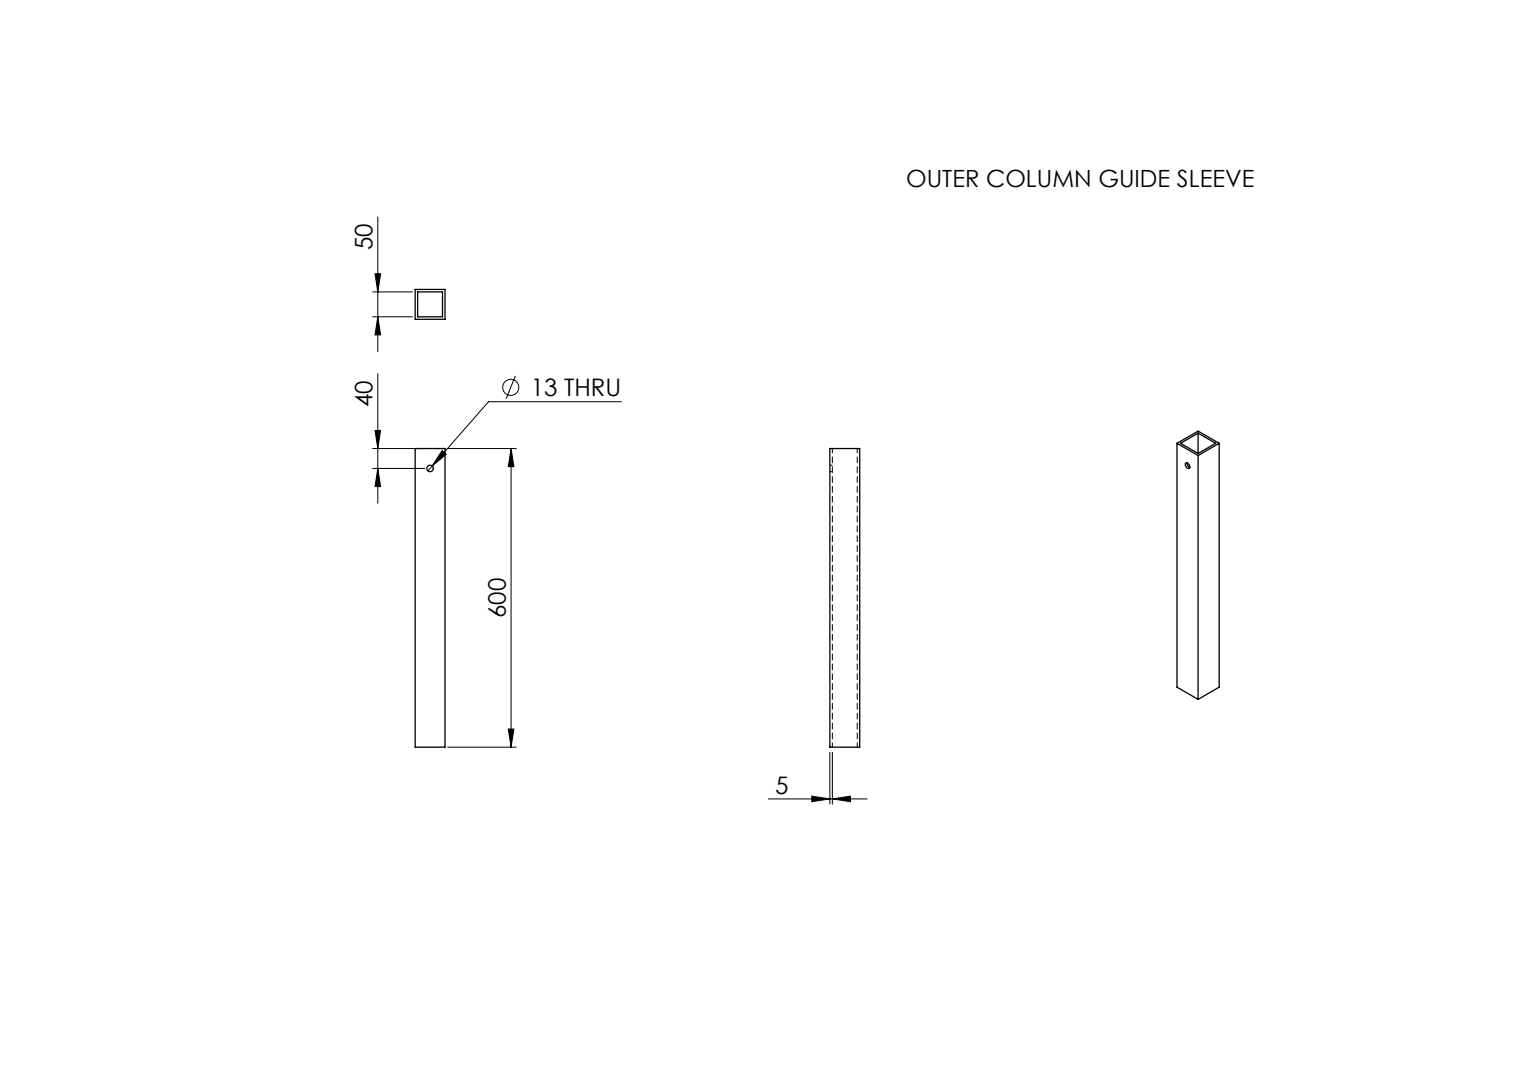
ISO-10303-21;
HEADER;
FILE_DESCRIPTION (('STEP AP214'),
    '1' );
FILE_NAME ('Outer Column Guide Sleeve.step',
    '2026-10-22T16:49:52',
    ( '' ),
    ( '' ),
    'SwSTEP 2.0',
    'SolidWorks 2026',
    '' );
FILE_SCHEMA (( 'AUTOMOTIVE_DESIGN' ));
ENDSEC;

DATA;
#4=( LENGTH_UNIT ( ) NAMED_UNIT ( * ) SI_UNIT ( .MILLI., .METRE. ) );
#55=DIRECTION ( 'NONE',  ( 0.000000000000000000, -0.000000000000000000, 1.000000000000000000 ) ) ;
#57=LINE ( 'NONE', #1683, #3118 ) ;
#59=CIRCLE ( 'NONE', #3730, 6.499999999999983125 ) ;
#64=DIRECTION ( 'NONE',  ( -0.000000000000000000, -0.000000000000000000, 1.000000000000000000 ) ) ;
#65=LINE ( 'NONE', #137, #1780 ) ;
#71=EDGE_LOOP ( 'NONE', ( #1973, #4142, #2111, #5305 ) ) ;
#74=DIRECTION ( 'NONE',  ( 1.000000000000000000, 0.000000000000000000, 0.000000000000000000 ) ) ;
#78=DIRECTION ( 'NONE',  ( -6.938893903907228378E-17, 0.000000000000000000, 1.000000000000000000 ) ) ;
#82=ORIENTED_EDGE ( 'NONE', *, *, #2566, .T. ) ;
#104=MANIFOLD_SOLID_BREP ( 'M12 Clearance Hole1', #2049 ) ;
#118=CIRCLE ( 'NONE', #3006, 6.499999999999988454 ) ;
#134=CARTESIAN_POINT ( 'NONE',  ( 30.00000000000000355, 610.0000000000000000, 30.00000000000001066 ) ) ;
#137=CARTESIAN_POINT ( 'NONE',  ( -24.99999999999999645, 610.0000000000000000, -25.00000000000000000 ) ) ;
#144=CARTESIAN_POINT ( 'NONE',  ( 0.000000000000000000, 570.0000000000000000, 25.00000000000000000 ) ) ;
#145=VECTOR ( 'NONE', #5158, 1000.000000000000000 ) ;
#150=VECTOR ( 'NONE', #4769, 1000.000000000000000 ) ;
#169=ORIENTED_EDGE ( 'NONE', *, *, #1169, .T. ) ;
#177=ORIENTED_EDGE ( 'NONE', *, *, #2712, .T. ) ;
#203=DIRECTION ( 'NONE',  ( 0.000000000000000000, 0.000000000000000000, -1.000000000000000000 ) ) ;
#213=DIRECTION ( 'NONE',  ( -1.000000000000000000, 0.000000000000000000, -2.081668171172168513E-16 ) ) ;
#220=ORIENTED_EDGE ( 'NONE', *, *, #4751, .F. ) ;
#236=CYLINDRICAL_SURFACE ( 'NONE', #2573, 6.499999999999983125 ) ;
#257=CARTESIAN_POINT ( 'NONE',  ( 30.00000000000000355, 610.0000000000000000, 30.00000000000001066 ) ) ;
#293=FACE_OUTER_BOUND ( 'NONE', #4919, .T. ) ;
#296=ORIENTED_EDGE ( 'NONE', *, *, #4163, .F. ) ;
#299=DIRECTION ( 'NONE',  ( -0.000000000000000000, -0.000000000000000000, 1.000000000000000000 ) ) ;
#306=DIRECTION ( 'NONE',  ( 1.000000000000000000, 0.000000000000000000, -0.000000000000000000 ) ) ;
#311=DIRECTION ( 'NONE',  ( -0.000000000000000000, -0.000000000000000000, 1.000000000000000000 ) ) ;
#324=EDGE_LOOP ( 'NONE', ( #2487, #2510, #2629, #3709 ) ) ;
#333=DIRECTION ( 'NONE',  ( -0.000000000000000000, -0.000000000000000000, 1.000000000000000000 ) ) ;
#337=FACE_OUTER_BOUND ( 'NONE', #718, .T. ) ;
#345=CARTESIAN_POINT ( 'NONE',  ( 30.00000000000000355, 610.0000000000000000, 0.000000000000000000 ) ) ;
#347=ORIENTED_EDGE ( 'NONE', *, *, #1984, .F. ) ;
#348=EDGE_LOOP ( 'NONE', ( #4253, #4137 ) ) ;
#363=FACE_BOUND ( 'NONE', #348, .T. ) ;
#384=ORIENTED_EDGE ( 'NONE', *, *, #564, .F. ) ;
#386=CARTESIAN_POINT ( 'NONE',  ( -30.00000000000000355, 610.0000000000000000, -2.081668171172168908E-15 ) ) ;
#401=( GEOMETRIC_REPRESENTATION_CONTEXT ( 3 ) GLOBAL_UNCERTAINTY_ASSIGNED_CONTEXT ( ( #3253 ) ) GLOBAL_UNIT_ASSIGNED_CONTEXT ( ( #4, #2110, #4596 ) ) REPRESENTATION_CONTEXT ( 'NONE', 'WORKASPACE' ) );
#441=CARTESIAN_POINT ( 'NONE',  ( -1.676835913137321903E-15, 35.00000000000000000, -25.00000000000000000 ) ) ;
#445=ORIENTED_EDGE ( 'NONE', *, *, #3007, .T. ) ;
#474=ORIENTED_EDGE ( 'NONE', *, *, #2211, .F. ) ;
#494=VECTOR ( 'NONE', #4759, 1000.000000000000000 ) ;
#502=AXIS2_PLACEMENT_3D ( 'NONE', #1265, #2612, #74 ) ;
#505=DIRECTION ( 'NONE',  ( -0.000000000000000000, -0.000000000000000000, 1.000000000000000000 ) ) ;
#516=DIRECTION ( 'NONE',  ( -0.000000000000000000, -1.000000000000000000, -0.000000000000000000 ) ) ;
#522=LINE ( 'NONE', #1310, #5104 ) ;
#525=ORIENTED_EDGE ( 'NONE', *, *, #1984, .T. ) ;
#528=CARTESIAN_POINT ( 'NONE',  ( -24.99999999999999645, 610.0000000000000000, -25.00000000000000000 ) ) ;
#536=DIRECTION ( 'NONE',  ( -0.000000000000000000, -0.000000000000000000, 1.000000000000000000 ) ) ;
#554=CARTESIAN_POINT ( 'NONE',  ( -1.676835913137321903E-15, 35.00000000000000000, 30.00000000000000711 ) ) ;
#555=CIRCLE ( 'NONE', #1685, 6.499999999999983125 ) ;
#564=EDGE_CURVE ( 'NONE', #1204, #676, #3614, .T. ) ;
#568=ORIENTED_EDGE ( 'NONE', *, *, #2743, .T. ) ;
#591=CARTESIAN_POINT ( 'NONE',  ( 0.000000000000000000, 570.0000000000000000, 25.00000000000000000 ) ) ;
#615=EDGE_LOOP ( 'NONE', ( #2413, #3333, #5322, #568 ) ) ;
#635=ORIENTED_EDGE ( 'NONE', *, *, #2387, .T. ) ;
#639=ORIENTED_EDGE ( 'NONE', *, *, #709, .F. ) ;
#652=VECTOR ( 'NONE', #4092, 1000.000000000000000 ) ;
#659=CARTESIAN_POINT ( 'NONE',  ( -24.99999999999999645, 610.0000000000000000, -25.00000000000000000 ) ) ;
#674=EDGE_LOOP ( 'NONE', ( #474, #4449, #1677, #4999 ) ) ;
#676=VERTEX_POINT ( 'NONE', #2760 ) ;
#680=VECTOR ( 'NONE', #5152, 1000.000000000000000 ) ;
#681=ORIENTED_EDGE ( 'NONE', *, *, #2414, .T. ) ;
#684=CARTESIAN_POINT ( 'NONE',  ( -30.00000000000000000, 610.0000000000000000, -30.00000000000000355 ) ) ;
#706=DIRECTION ( 'NONE',  ( 0.000000000000000000, -0.000000000000000000, 1.000000000000000000 ) ) ;
#709=EDGE_CURVE ( 'NONE', #819, #4789, #1060, .T. ) ;
#714=DIRECTION ( 'NONE',  ( -1.000000000000000000, 0.000000000000000000, -0.000000000000000000 ) ) ;
#718=EDGE_LOOP ( 'NONE', ( #2881, #2906, #4894, #4616 ) ) ;
#722=LINE ( 'NONE', #5277, #1209 ) ;
#734=AXIS2_PLACEMENT_3D ( 'NONE', #3221, #1943, #706 ) ;
#735=ORIENTED_EDGE ( 'NONE', *, *, #1905, .T. ) ;
#751=COLOUR_RGB ( '',0.8941176470588234615, 0.8941176470588234615, 0.8941176470588234615 ) ;
#761=VECTOR ( 'NONE', #2328, 1000.000000000000000 ) ;
#767=ORIENTED_EDGE ( 'NONE', *, *, #3722, .F. ) ;
#769=DIRECTION ( 'NONE',  ( 1.000000000000000000, 0.000000000000000000, 0.000000000000000000 ) ) ;
#776=DIRECTION ( 'NONE',  ( 1.000000000000000000, 0.000000000000000000, 0.000000000000000000 ) ) ;
#797=CARTESIAN_POINT ( 'NONE',  ( 25.00000000000000000, 610.0000000000000000, 25.00000000000000711 ) ) ;
#819=VERTEX_POINT ( 'NONE', #797 ) ;
#823=DIRECTION ( 'NONE',  ( -1.000000000000000000, 0.000000000000000000, 0.000000000000000000 ) ) ;
#834=LINE ( 'NONE', #4115, #1093 ) ;
#840=PRODUCT_DEFINITION_FORMATION_WITH_SPECIFIED_SOURCE ( 'ANY', '', #918, .NOT_KNOWN. ) ;
#845=FILL_AREA_STYLE ('',( #3720 ) ) ;
#851=EDGE_LOOP ( 'NONE', ( #978, #1701, #2976, #2915 ) ) ;
#858=CARTESIAN_POINT ( 'NONE',  ( 0.000000000000000000, 570.0000000000000000, 30.00000000000000711 ) ) ;
#868=FACE_OUTER_BOUND ( 'NONE', #5245, .T. ) ;
#890=CARTESIAN_POINT ( 'NONE',  ( -1.676835913137321903E-15, 35.00000000000000000, -30.00000000000000711 ) ) ;
#911=ADVANCED_FACE ( 'NONE', ( #2175 ), #2619, .T. ) ;
#918=PRODUCT ( 'Outer Column Guide Sleeve', 'Outer Column Guide Sleeve', '', ( #3228 ) ) ;
#927=ORIENTED_EDGE ( 'NONE', *, *, #4973, .F. ) ;
#933=( NAMED_UNIT ( * ) SI_UNIT ( $, .STERADIAN. ) SOLID_ANGLE_UNIT ( ) );
#939=DIRECTION ( 'NONE',  ( -0.000000000000000000, -0.000000000000000000, 1.000000000000000000 ) ) ;
#966=VERTEX_POINT ( 'NONE', #3415 ) ;
#969=CARTESIAN_POINT ( 'NONE',  ( 25.00000000000000000, 610.0000000000000000, 25.00000000000000711 ) ) ;
#978=ORIENTED_EDGE ( 'NONE', *, *, #1193, .T. ) ;
#984=LINE ( 'NONE', #1407, #145 ) ;
#995=DIRECTION ( 'NONE',  ( -0.000000000000000000, -1.000000000000000000, -0.000000000000000000 ) ) ;
#1021=EDGE_CURVE ( 'NONE', #1591, #4832, #555, .T. ) ;
#1038=DIRECTION ( 'NONE',  ( 0.000000000000000000, 0.000000000000000000, -1.000000000000000000 ) ) ;
#1040=PLANE ( 'NONE',  #3295 ) ;
#1049=CARTESIAN_POINT ( 'NONE',  ( -30.00000000000000355, 610.0000000000000000, 30.00000000000000000 ) ) ;
#1054=ORIENTED_EDGE ( 'NONE', *, *, #4694, .T. ) ;
#1060=LINE ( 'NONE', #4411, #5259 ) ;
#1061=LINE ( 'NONE', #2731, #2423 ) ;
#1062=FACE_BOUND ( 'NONE', #2196, .T. ) ;
#1065=SHAPE_REPRESENTATION ( 'Outer Column Guide Sleeve', ( #4154 ), #3189 ) ;
#1066=EDGE_CURVE ( 'NONE', #2454, #4719, #118, .T. ) ;
#1069=CARTESIAN_POINT ( 'NONE',  ( 30.00000000000000355, 610.0000000000000000, 0.000000000000000000 ) ) ;
#1074=CARTESIAN_POINT ( 'NONE',  ( -25.00000000000000000, 610.0000000000000000, 24.99999999999999645 ) ) ;
#1075=VERTEX_POINT ( 'NONE', #5044 ) ;
#1093=VECTOR ( 'NONE', #4947, 1000.000000000000000 ) ;
#1101=AXIS2_PLACEMENT_3D ( 'NONE', #1578, #5333, #3322 ) ;
#1105=FACE_OUTER_BOUND ( 'NONE', #71, .T. ) ;
#1109=EDGE_CURVE ( 'NONE', #3821, #4454, #1453, .T. ) ;
#1122=UNCERTAINTY_MEASURE_WITH_UNIT (LENGTH_MEASURE( 1.000000000000000082E-05 ), #3066, 'distance_accuracy_value', 'NONE');
#1124=EDGE_LOOP ( 'NONE', ( #2187, #2700, #3235, #525 ) ) ;
#1125=PLANE ( 'NONE',  #3717 ) ;
#1138=PLANE ( 'NONE',  #734 ) ;
#1169=EDGE_CURVE ( 'NONE', #4363, #3498, #2834, .T. ) ;
#1193=EDGE_CURVE ( 'NONE', #1510, #1969, #3155, .T. ) ;
#1199=CARTESIAN_POINT ( 'NONE',  ( 30.00000000000000355, 10.00000000000000000, -30.00000000000000355 ) ) ;
#1203=( NAMED_UNIT ( * ) PLANE_ANGLE_UNIT ( ) SI_UNIT ( $, .RADIAN. ) );
#1204=VERTEX_POINT ( 'NONE', #1393 ) ;
#1209=VECTOR ( 'NONE', #311, 1000.000000000000000 ) ;
#1228=SHAPE_REPRESENTATION_RELATIONSHIP ( 'NONE' , 'NONE' ,  #1065, #4286 ) ;
#1241=EDGE_CURVE ( 'NONE', #4454, #966, #3104, .T. ) ;
#1249=EDGE_LOOP ( 'NONE', ( #767, #2867, #5272, #681 ) ) ;
#1265=CARTESIAN_POINT ( 'NONE',  ( -1.676835913137321903E-15, 35.00000000000000000, -25.00000000000000000 ) ) ;
#1275=ADVANCED_FACE ( 'NONE', ( #5288, #4865 ), #1138, .T. ) ;
#1283=AXIS2_PLACEMENT_3D ( 'NONE', #3128, #4799, #3416 ) ;
#1285=ORIENTED_EDGE ( 'NONE', *, *, #3872, .F. ) ;
#1294=ORIENTED_EDGE ( 'NONE', *, *, #4878, .T. ) ;
#1310=CARTESIAN_POINT ( 'NONE',  ( -6.245004513516506329E-15, 610.0000000000000000, 30.00000000000000711 ) ) ;
#1317=DIRECTION ( 'NONE',  ( 1.000000000000000000, 0.000000000000000000, 0.000000000000000000 ) ) ;
#1348=DIRECTION ( 'NONE',  ( -0.000000000000000000, -1.000000000000000000, -0.000000000000000000 ) ) ;
#1358=DIRECTION ( 'NONE',  ( -1.000000000000000000, 0.000000000000000000, 0.000000000000000000 ) ) ;
#1366=DIRECTION ( 'NONE',  ( -1.000000000000000000, 0.000000000000000000, 0.000000000000000000 ) ) ;
#1374=DIRECTION ( 'NONE',  ( 6.938893903907228378E-17, 0.000000000000000000, -1.000000000000000000 ) ) ;
#1384=DIRECTION ( 'NONE',  ( 2.081668171172168513E-16, 0.000000000000000000, -1.000000000000000000 ) ) ;
#1393=CARTESIAN_POINT ( 'NONE',  ( -6.499999999999984901, 35.00000000000000000, 25.00000000000000000 ) ) ;
#1397=VERTEX_POINT ( 'NONE', #2602 ) ;
#1407=CARTESIAN_POINT ( 'NONE',  ( 30.00000000000000355, 610.0000000000000000, -30.00000000000000355 ) ) ;
#1410=FACE_OUTER_BOUND ( 'NONE', #1249, .T. ) ;
#1414=VECTOR ( 'NONE', #1348, 1000.000000000000000 ) ;
#1453=LINE ( 'NONE', #2226, #3873 ) ;
#1457=VERTEX_POINT ( 'NONE', #4315 ) ;
#1468=CARTESIAN_POINT ( 'NONE',  ( 25.00000000000000000, 10.00000000000000000, -25.00000000000000000 ) ) ;
#1478=EDGE_LOOP ( 'NONE', ( #4056, #1960 ) ) ;
#1483=ORIENTED_EDGE ( 'NONE', *, *, #3142, .T. ) ;
#1503=AXIS2_PLACEMENT_3D ( 'NONE', #591, #3185, #4780 ) ;
#1509=ADVANCED_FACE ( 'NONE', ( #5106, #2689 ), #4345, .F. ) ;
#1510=VERTEX_POINT ( 'NONE', #5156 ) ;
#1511=VECTOR ( 'NONE', #78, 1000.000000000000000 ) ;
#1532=ORIENTED_EDGE ( 'NONE', *, *, #5162, .T. ) ;
#1534=VECTOR ( 'NONE', #4371, 1000.000000000000000 ) ;
#1578=CARTESIAN_POINT ( 'NONE',  ( -6.245004513516506329E-15, 610.0000000000000000, 30.00000000000000711 ) ) ;
#1591=VERTEX_POINT ( 'NONE', #3674 ) ;
#1601=AXIS2_PLACEMENT_3D ( 'NONE', #3718, #3746, #5371 ) ;
#1619=AXIS2_PLACEMENT_3D ( 'NONE', #386, #2917, #2497 ) ;
#1626=( LENGTH_UNIT ( ) NAMED_UNIT ( * ) SI_UNIT ( .MILLI., .METRE. ) );
#1653=ADVANCED_FACE ( 'NONE', ( #4851, #337 ), #1125, .F. ) ;
#1657=ORIENTED_EDGE ( 'NONE', *, *, #5072, .T. ) ;
#1665=( GEOMETRIC_REPRESENTATION_CONTEXT ( 3 ) GLOBAL_UNCERTAINTY_ASSIGNED_CONTEXT ( ( #1122 ) ) GLOBAL_UNIT_ASSIGNED_CONTEXT ( ( #3066, #4242, #933 ) ) REPRESENTATION_CONTEXT ( 'NONE', 'WORKASPACE' ) );
#1677=ORIENTED_EDGE ( 'NONE', *, *, #4751, .T. ) ;
#1678=ORIENTED_EDGE ( 'NONE', *, *, #3048, .T. ) ;
#1683=CARTESIAN_POINT ( 'NONE',  ( 6.499999999999981348, 35.00000000000000000, 30.00000000000000711 ) ) ;
#1685=AXIS2_PLACEMENT_3D ( 'NONE', #890, #55, #4643 ) ;
#1688=AXIS2_PLACEMENT_3D ( 'NONE', #4682, #1828, #4287 ) ;
#1690=FACE_OUTER_BOUND ( 'NONE', #2461, .T. ) ;
#1697=PLANE ( 'NONE',  #2774 ) ;
#1701=ORIENTED_EDGE ( 'NONE', *, *, #3430, .F. ) ;
#1713=DIRECTION ( 'NONE',  ( 1.000000000000000000, 0.000000000000000000, 0.000000000000000000 ) ) ;
#1718=EDGE_CURVE ( 'NONE', #4147, #4026, #4642, .T. ) ;
#1727=AXIS2_PLACEMENT_3D ( 'NONE', #2764, #333, #4108 ) ;
#1750=STYLED_ITEM('',(#5440),#104);
#1758=CARTESIAN_POINT ( 'NONE',  ( -25.00000000000000000, 610.0000000000000000, 24.99999999999999645 ) ) ;
#1765=CARTESIAN_POINT ( 'NONE',  ( -1.676835913137321903E-15, 35.00000000000000000, 25.00000000000000000 ) ) ;
#1770=ORIENTED_EDGE ( 'NONE', *, *, #1109, .T. ) ;
#1780=VECTOR ( 'NONE', #1825, 1000.000000000000000 ) ;
#1801=ORIENTED_EDGE ( 'NONE', *, *, #4432, .T. ) ;
#1815=ADVANCED_FACE ( 'NONE', ( #4330 ), #236, .F. ) ;
#1823=DIRECTION ( 'NONE',  ( -1.000000000000000000, 0.000000000000000000, 0.000000000000000000 ) ) ;
#1825=DIRECTION ( 'NONE',  ( -1.000000000000000000, 0.000000000000000000, -0.000000000000000000 ) ) ;
#1828=DIRECTION ( 'NONE',  ( 0.000000000000000000, 1.000000000000000000, 0.000000000000000000 ) ) ;
#1872=CARTESIAN_POINT ( 'NONE',  ( 6.499999999999981348, 35.00000000000000000, -30.00000000000000711 ) ) ;
#1883=CARTESIAN_POINT ( 'NONE',  ( -6.499999999999984901, 35.00000000000000000, -25.00000000000000000 ) ) ;
#1890=VECTOR ( 'NONE', #516, 1000.000000000000000 ) ;
#1895=CARTESIAN_POINT ( 'NONE',  ( 0.000000000000000000, 570.0000000000000000, 30.00000000000000711 ) ) ;
#1903=DIRECTION ( 'NONE',  ( 1.000000000000000000, 0.000000000000000000, 0.000000000000000000 ) ) ;
#1905=EDGE_CURVE ( 'NONE', #4719, #2454, #3093, .T. ) ;
#1924=DIRECTION ( 'NONE',  ( 1.000000000000000000, 0.000000000000000000, 2.081668171172168513E-16 ) ) ;
#1942=ORIENTED_EDGE ( 'NONE', *, *, #3391, .F. ) ;
#1943=DIRECTION ( 'NONE',  ( 0.000000000000000000, 1.000000000000000000, 0.000000000000000000 ) ) ;
#1954=PRODUCT_DEFINITION_SHAPE ( 'NONE', 'NONE',  #4133 ) ;
#1960=ORIENTED_EDGE ( 'NONE', *, *, #3022, .F. ) ;
#1969=VERTEX_POINT ( 'NONE', #1199 ) ;
#1973=ORIENTED_EDGE ( 'NONE', *, *, #4694, .F. ) ;
#1982=CARTESIAN_POINT ( 'NONE',  ( 6.499999999999993783, 570.0000000000000000, 30.00000000000000711 ) ) ;
#1984=EDGE_CURVE ( 'NONE', #4026, #3218, #2480, .T. ) ;
#1990=UNCERTAINTY_MEASURE_WITH_UNIT (LENGTH_MEASURE( 1.000000000000000082E-05 ), #1626, 'distance_accuracy_value', 'NONE');
#1991=SHAPE_DEFINITION_REPRESENTATION ( #1954, #1065 ) ;
#1995=EDGE_LOOP ( 'NONE', ( #3331, #639, #1285, #220 ) ) ;
#1998=DIRECTION ( 'NONE',  ( 0.000000000000000000, 0.000000000000000000, 1.000000000000000000 ) ) ;
#2012=ORIENTED_EDGE ( 'NONE', *, *, #1241, .F. ) ;
#2033=ORIENTED_EDGE ( 'NONE', *, *, #3007, .F. ) ;
#2049=CLOSED_SHELL ( 'NONE', ( #1815, #2075, #5383, #2874, #1275, #1509, #4252, #1653, #3658, #4584, #4343, #911, #3183, #4050, #2401, #4954 ) ) ;
#2062=ORIENTED_EDGE ( 'NONE', *, *, #5162, .F. ) ;
#2075=ADVANCED_FACE ( 'NONE', ( #868 ), #3866, .F. ) ;
#2086=EDGE_LOOP ( 'NONE', ( #927, #2033 ) ) ;
#2094=DIRECTION ( 'NONE',  ( -0.000000000000000000, -1.000000000000000000, -0.000000000000000000 ) ) ;
#2110=( NAMED_UNIT ( * ) PLANE_ANGLE_UNIT ( ) SI_UNIT ( $, .RADIAN. ) );
#2111=ORIENTED_EDGE ( 'NONE', *, *, #5360, .T. ) ;
#2166=CARTESIAN_POINT ( 'NONE',  ( 6.499999999999993783, 570.0000000000000000, 25.00000000000000000 ) ) ;
#2167=APPLICATION_CONTEXT ( 'automotive_design' ) ;
#2175=FACE_OUTER_BOUND ( 'NONE', #674, .T. ) ;
#2184=CARTESIAN_POINT ( 'NONE',  ( 6.499999999999986677, 35.00000000000000000, 30.00000000000000711 ) ) ;
#2187=ORIENTED_EDGE ( 'NONE', *, *, #3722, .T. ) ;
#2189=EDGE_LOOP ( 'NONE', ( #2549, #4188, #2720, #296 ) ) ;
#2196=EDGE_LOOP ( 'NONE', ( #1942, #384 ) ) ;
#2211=EDGE_CURVE ( 'NONE', #2280, #4026, #3387, .T. ) ;
#2222=VECTOR ( 'NONE', #2842, 1000.000000000000000 ) ;
#2226=CARTESIAN_POINT ( 'NONE',  ( -30.00000000000000355, 610.0000000000000000, -2.081668171172168908E-15 ) ) ;
#2259=ORIENTED_EDGE ( 'NONE', *, *, #4401, .T. ) ;
#2262=FACE_BOUND ( 'NONE', #3264, .T. ) ;
#2271=DIRECTION ( 'NONE',  ( -1.000000000000000000, 0.000000000000000000, 0.000000000000000000 ) ) ;
#2280=VERTEX_POINT ( 'NONE', #2664 ) ;
#2290=FACE_OUTER_BOUND ( 'NONE', #2869, .T. ) ;
#2318=LINE ( 'NONE', #3552, #4927 ) ;
#2319=CARTESIAN_POINT ( 'NONE',  ( -1.676835913137321903E-15, 35.00000000000000000, 30.00000000000000711 ) ) ;
#2322=AXIS2_PLACEMENT_3D ( 'NONE', #144, #1384, #1366 ) ;
#2328=DIRECTION ( 'NONE',  ( -0.000000000000000000, -1.000000000000000000, -0.000000000000000000 ) ) ;
#2345=ORIENTED_EDGE ( 'NONE', *, *, #1169, .F. ) ;
#2387=EDGE_CURVE ( 'NONE', #1591, #2639, #4557, .T. ) ;
#2401=ADVANCED_FACE ( 'NONE', ( #3236 ), #3683, .F. ) ;
#2413=ORIENTED_EDGE ( 'NONE', *, *, #5071, .F. ) ;
#2414=EDGE_CURVE ( 'NONE', #4789, #4512, #834, .T. ) ;
#2423=VECTOR ( 'NONE', #1924, 1000.000000000000000 ) ;
#2434=CARTESIAN_POINT ( 'NONE',  ( 0.000000000000000000, 0.000000000000000000, 0.000000000000000000 ) ) ;
#2447=FACE_OUTER_BOUND ( 'NONE', #324, .T. ) ;
#2450=CARTESIAN_POINT ( 'NONE',  ( -1.676835913137321903E-15, 35.00000000000000000, 30.00000000000000711 ) ) ;
#2454=VERTEX_POINT ( 'NONE', #5279 ) ;
#2461=EDGE_LOOP ( 'NONE', ( #1801, #2012, #3367, #4779 ) ) ;
#2480=LINE ( 'NONE', #2512, #3721 ) ;
#2487=ORIENTED_EDGE ( 'NONE', *, *, #4218, .T. ) ;
#2497=DIRECTION ( 'NONE',  ( 6.938893903907228378E-17, 0.000000000000000000, -1.000000000000000000 ) ) ;
#2510=ORIENTED_EDGE ( 'NONE', *, *, #3208, .F. ) ;
#2512=CARTESIAN_POINT ( 'NONE',  ( -25.00000000000000000, 10.00000000000000000, 24.99999999999999645 ) ) ;
#2549=ORIENTED_EDGE ( 'NONE', *, *, #1193, .F. ) ;
#2566=EDGE_CURVE ( 'NONE', #4832, #4261, #4291, .T. ) ;
#2573=AXIS2_PLACEMENT_3D ( 'NONE', #3101, #4431, #3630 ) ;
#2575=LINE ( 'NONE', #4281, #5197 ) ;
#2586=DIRECTION ( 'NONE',  ( -0.000000000000000000, 0.000000000000000000, 1.000000000000000000 ) ) ;
#2588=ORIENTED_EDGE ( 'NONE', *, *, #1021, .T. ) ;
#2594=CARTESIAN_POINT ( 'NONE',  ( -1.676835913137321903E-15, 35.00000000000000000, 30.00000000000000711 ) ) ;
#2602=CARTESIAN_POINT ( 'NONE',  ( -30.00000000000000000, 10.00000000000000000, -30.00000000000000355 ) ) ;
#2612=DIRECTION ( 'NONE',  ( -0.000000000000000000, 0.000000000000000000, 1.000000000000000000 ) ) ;
#2619=PLANE ( 'NONE',  #3434 ) ;
#2629=ORIENTED_EDGE ( 'NONE', *, *, #3048, .F. ) ;
#2639=VERTEX_POINT ( 'NONE', #1883 ) ;
#2642=DIRECTION ( 'NONE',  ( 1.000000000000000000, -0.000000000000000000, 6.938893903907228378E-17 ) ) ;
#2650=CARTESIAN_POINT ( 'NONE',  ( -6.499999999999984901, 35.00000000000000000, 30.00000000000000711 ) ) ;
#2664=CARTESIAN_POINT ( 'NONE',  ( -24.99999999999999645, 10.00000000000000000, -25.00000000000000000 ) ) ;
#2679=AXIS2_PLACEMENT_3D ( 'NONE', #4544, #3315, #823 ) ;
#2688=VECTOR ( 'NONE', #2900, 1000.000000000000000 ) ;
#2689=FACE_BOUND ( 'NONE', #1124, .T. ) ;
#2694=CIRCLE ( 'NONE', #1727, 6.499999999999988454 ) ;
#2700=ORIENTED_EDGE ( 'NONE', *, *, #5071, .T. ) ;
#2712=EDGE_CURVE ( 'NONE', #4028, #1457, #3915, .T. ) ;
#2720=ORIENTED_EDGE ( 'NONE', *, *, #4432, .F. ) ;
#2725=CARTESIAN_POINT ( 'NONE',  ( 30.00000000000000355, 10.00000000000000000, 0.000000000000000000 ) ) ;
#2731=CARTESIAN_POINT ( 'NONE',  ( -25.00000000000000000, 610.0000000000000000, 24.99999999999999645 ) ) ;
#2743=EDGE_CURVE ( 'NONE', #5225, #2280, #4393, .T. ) ;
#2760=CARTESIAN_POINT ( 'NONE',  ( 6.499999999999981348, 35.00000000000000000, 25.00000000000000000 ) ) ;
#2764=CARTESIAN_POINT ( 'NONE',  ( 0.000000000000000000, 570.0000000000000000, 30.00000000000000711 ) ) ;
#2774=AXIS2_PLACEMENT_3D ( 'NONE', #528, #2586, #1317 ) ;
#2785=DIRECTION ( 'NONE',  ( 1.000000000000000000, 0.000000000000000000, 0.000000000000000000 ) ) ;
#2800=DIRECTION ( 'NONE',  ( 1.000000000000000000, 0.000000000000000000, 0.000000000000000000 ) ) ;
#2820=DIRECTION ( 'NONE',  ( 0.000000000000000000, -0.000000000000000000, 1.000000000000000000 ) ) ;
#2824=PRODUCT_DEFINITION_CONTEXT ( 'detailed design', #5061, 'design' ) ;
#2831=ORIENTED_EDGE ( 'NONE', *, *, #3391, .T. ) ;
#2834=CIRCLE ( 'NONE', #1503, 6.499999999999993783 ) ;
#2837=EDGE_LOOP ( 'NONE', ( #347, #3969, #3702, #3549 ) ) ;
#2842=DIRECTION ( 'NONE',  ( -0.000000000000000000, -0.000000000000000000, 1.000000000000000000 ) ) ;
#2867=ORIENTED_EDGE ( 'NONE', *, *, #5214, .F. ) ;
#2869=EDGE_LOOP ( 'NONE', ( #3781, #3510, #1532, #735 ) ) ;
#2874=ADVANCED_FACE ( 'NONE', ( #363, #2447, #4059 ), #4134, .F. ) ;
#2881=ORIENTED_EDGE ( 'NONE', *, *, #4163, .T. ) ;
#2900=DIRECTION ( 'NONE',  ( 1.000000000000000000, 0.000000000000000000, 2.081668171172168513E-16 ) ) ;
#2906=ORIENTED_EDGE ( 'NONE', *, *, #3921, .F. ) ;
#2915=ORIENTED_EDGE ( 'NONE', *, *, #3208, .T. ) ;
#2917=DIRECTION ( 'NONE',  ( 1.000000000000000000, -0.000000000000000000, 6.938893903907228378E-17 ) ) ;
#2918=DIRECTION ( 'NONE',  ( 1.000000000000000000, 0.000000000000000000, 0.000000000000000000 ) ) ;
#2924=DIRECTION ( 'NONE',  ( 0.000000000000000000, 0.000000000000000000, 1.000000000000000000 ) ) ;
#2976=ORIENTED_EDGE ( 'NONE', *, *, #2712, .F. ) ;
#2989=DIRECTION ( 'NONE',  ( 1.000000000000000000, 0.000000000000000000, 2.081668171172168513E-16 ) ) ;
#3006=AXIS2_PLACEMENT_3D ( 'NONE', #2594, #536, #1713 ) ;
#3007=EDGE_CURVE ( 'NONE', #1075, #4782, #3890, .T. ) ;
#3022=EDGE_CURVE ( 'NONE', #2639, #4261, #59, .T. ) ;
#3048=EDGE_CURVE ( 'NONE', #4454, #4028, #522, .T. ) ;
#3066=( LENGTH_UNIT ( ) NAMED_UNIT ( * ) SI_UNIT ( .MILLI., .METRE. ) );
#3072=ORIENTED_EDGE ( 'NONE', *, *, #5072, .F. ) ;
#3092=LINE ( 'NONE', #4004, #150 ) ;
#3093=CIRCLE ( 'NONE', #1601, 6.499999999999988454 ) ;
#3101=CARTESIAN_POINT ( 'NONE',  ( -1.676835913137321903E-15, 35.00000000000000000, 30.00000000000000711 ) ) ;
#3104=LINE ( 'NONE', #4839, #3358 ) ;
#3115=LINE ( 'NONE', #2650, #680 ) ;
#3118=VECTOR ( 'NONE', #3363, 1000.000000000000000 ) ;
#3128=CARTESIAN_POINT ( 'NONE',  ( 0.000000000000000000, 570.0000000000000000, 30.00000000000000711 ) ) ;
#3142=EDGE_CURVE ( 'NONE', #1457, #3821, #2318, .T. ) ;
#3149=ORIENTED_EDGE ( 'NONE', *, *, #3022, .T. ) ;
#3155=LINE ( 'NONE', #2725, #3269 ) ;
#3174=LINE ( 'NONE', #4831, #1534 ) ;
#3183=ADVANCED_FACE ( 'NONE', ( #1062, #2262, #3958 ), #1040, .T. ) ;
#3185=DIRECTION ( 'NONE',  ( 2.081668171172168513E-16, 0.000000000000000000, -1.000000000000000000 ) ) ;
#3189=( GEOMETRIC_REPRESENTATION_CONTEXT ( 3 ) GLOBAL_UNCERTAINTY_ASSIGNED_CONTEXT ( ( #1990 ) ) GLOBAL_UNIT_ASSIGNED_CONTEXT ( ( #1626, #1203, #3276 ) ) REPRESENTATION_CONTEXT ( 'NONE', 'WORKASPACE' ) );
#3208=EDGE_CURVE ( 'NONE', #4028, #1510, #5127, .T. ) ;
#3218=VERTEX_POINT ( 'NONE', #4360 ) ;
#3221=CARTESIAN_POINT ( 'NONE',  ( 0.000000000000000000, 610.0000000000000000, 0.000000000000000000 ) ) ;
#3228=PRODUCT_CONTEXT ( 'NONE', #2167, 'mechanical' ) ;
#3235=ORIENTED_EDGE ( 'NONE', *, *, #2211, .T. ) ;
#3236=FACE_OUTER_BOUND ( 'NONE', #3714, .T. ) ;
#3253=UNCERTAINTY_MEASURE_WITH_UNIT (LENGTH_MEASURE( 1.000000000000000082E-05 ), #4, 'distance_accuracy_value', 'NONE');
#3255=CARTESIAN_POINT ( 'NONE',  ( 0.000000000000000000, 610.0000000000000000, -30.00000000000000355 ) ) ;
#3264=EDGE_LOOP ( 'NONE', ( #2345, #4775 ) ) ;
#3268=EDGE_LOOP ( 'NONE', ( #2831, #1294, #5124, #2062 ) ) ;
#3269=VECTOR ( 'NONE', #203, 1000.000000000000000 ) ;
#3276=( NAMED_UNIT ( * ) SI_UNIT ( $, .STERADIAN. ) SOLID_ANGLE_UNIT ( ) );
#3295=AXIS2_PLACEMENT_3D ( 'NONE', #3932, #4677, #213 ) ;
#3296=CIRCLE ( 'NONE', #2322, 6.499999999999993783 ) ;
#3305=AXIS2_PLACEMENT_3D ( 'NONE', #4349, #2271, #1998 ) ;
#3315=DIRECTION ( 'NONE',  ( 2.081668171172168513E-16, 0.000000000000000000, -1.000000000000000000 ) ) ;
#3322=DIRECTION ( 'NONE',  ( -1.000000000000000000, 0.000000000000000000, -2.081668171172168513E-16 ) ) ;
#3331=ORIENTED_EDGE ( 'NONE', *, *, #4800, .F. ) ;
#3333=ORIENTED_EDGE ( 'NONE', *, *, #2414, .F. ) ;
#3343=DIRECTION ( 'NONE',  ( 1.000000000000000000, 0.000000000000000000, 0.000000000000000000 ) ) ;
#3358=VECTOR ( 'NONE', #995, 1000.000000000000000 ) ;
#3363=DIRECTION ( 'NONE',  ( -0.000000000000000000, -0.000000000000000000, 1.000000000000000000 ) ) ;
#3367=ORIENTED_EDGE ( 'NONE', *, *, #1109, .F. ) ;
#3387=LINE ( 'NONE', #3817, #1511 ) ;
#3390=SURFACE_STYLE_USAGE ( .BOTH. , #4219 ) ;
#3391=EDGE_CURVE ( 'NONE', #676, #1204, #5030, .T. ) ;
#3415=CARTESIAN_POINT ( 'NONE',  ( -30.00000000000000355, 10.00000000000000000, 30.00000000000000000 ) ) ;
#3416=DIRECTION ( 'NONE',  ( 1.000000000000000000, 0.000000000000000000, 0.000000000000000000 ) ) ;
#3424=CARTESIAN_POINT ( 'NONE',  ( -25.00000000000000000, 610.0000000000000000, 24.99999999999999645 ) ) ;
#3430=EDGE_CURVE ( 'NONE', #1457, #1969, #984, .T. ) ;
#3434=AXIS2_PLACEMENT_3D ( 'NONE', #3870, #2642, #1374 ) ;
#3444=DIRECTION ( 'NONE',  ( 2.081668171172168513E-16, 0.000000000000000000, -1.000000000000000000 ) ) ;
#3461=VECTOR ( 'NONE', #4707, 1000.000000000000000 ) ;
#3475=VECTOR ( 'NONE', #714, 1000.000000000000000 ) ;
#3498=VERTEX_POINT ( 'NONE', #5135 ) ;
#3506=EDGE_CURVE ( 'NONE', #3498, #4363, #3296, .T. ) ;
#3510=ORIENTED_EDGE ( 'NONE', *, *, #564, .T. ) ;
#3515=AXIS2_PLACEMENT_3D ( 'NONE', #1765, #3444, #1358 ) ;
#3549=ORIENTED_EDGE ( 'NONE', *, *, #5214, .T. ) ;
#3552=CARTESIAN_POINT ( 'NONE',  ( 0.000000000000000000, 610.0000000000000000, -30.00000000000000355 ) ) ;
#3553=CYLINDRICAL_SURFACE ( 'NONE', #4251, 6.499999999999983125 ) ;
#3575=DIRECTION ( 'NONE',  ( -0.000000000000000000, -0.000000000000000000, 1.000000000000000000 ) ) ;
#3614=CIRCLE ( 'NONE', #3515, 6.499999999999983125 ) ;
#3627=STYLED_ITEM ( 'NONE', ( #3748 ), #4286 ) ;
#3630=DIRECTION ( 'NONE',  ( 1.000000000000000000, 0.000000000000000000, 0.000000000000000000 ) ) ;
#3633=AXIS2_PLACEMENT_3D ( 'NONE', #345, #4034, #2924 ) ;
#3634=LINE ( 'NONE', #1982, #2222 ) ;
#3658=ADVANCED_FACE ( 'NONE', ( #1690 ), #4550, .F. ) ;
#3674=CARTESIAN_POINT ( 'NONE',  ( -6.499999999999984901, 35.00000000000000000, -30.00000000000000711 ) ) ;
#3683=CYLINDRICAL_SURFACE ( 'NONE', #3725, 6.499999999999983125 ) ;
#3702=ORIENTED_EDGE ( 'NONE', *, *, #3872, .T. ) ;
#3709=ORIENTED_EDGE ( 'NONE', *, *, #1241, .T. ) ;
#3714=EDGE_LOOP ( 'NONE', ( #4722, #3072, #82, #2259 ) ) ;
#3717=AXIS2_PLACEMENT_3D ( 'NONE', #3255, #2820, #306 ) ;
#3718=CARTESIAN_POINT ( 'NONE',  ( -1.676835913137321903E-15, 35.00000000000000000, 30.00000000000000711 ) ) ;
#3720=FILL_AREA_STYLE_COLOUR ( '', #751 ) ;
#3721=VECTOR ( 'NONE', #4145, 1000.000000000000000 ) ;
#3722=EDGE_CURVE ( 'NONE', #3218, #4512, #2575, .T. ) ;
#3725=AXIS2_PLACEMENT_3D ( 'NONE', #2450, #4976, #2800 ) ;
#3730=AXIS2_PLACEMENT_3D ( 'NONE', #441, #3777, #3343 ) ;
#3746=DIRECTION ( 'NONE',  ( -0.000000000000000000, -0.000000000000000000, 1.000000000000000000 ) ) ;
#3748=PRESENTATION_STYLE_ASSIGNMENT (( #3390 ) ) ;
#3777=DIRECTION ( 'NONE',  ( -0.000000000000000000, 0.000000000000000000, 1.000000000000000000 ) ) ;
#3781=ORIENTED_EDGE ( 'NONE', *, *, #4878, .F. ) ;
#3801=AXIS2_PLACEMENT_3D ( 'NONE', #1895, #3575, #2785 ) ;
#3817=CARTESIAN_POINT ( 'NONE',  ( -25.00000000000000000, 10.00000000000000000, 24.99999999999999645 ) ) ;
#3820=VECTOR ( 'NONE', #4234, 1000.000000000000000 ) ;
#3821=VERTEX_POINT ( 'NONE', #684 ) ;
#3864=FACE_OUTER_BOUND ( 'NONE', #615, .T. ) ;
#3866=CYLINDRICAL_SURFACE ( 'NONE', #5364, 6.499999999999983125 ) ;
#3870=CARTESIAN_POINT ( 'NONE',  ( -25.00000000000000000, 610.0000000000000000, 24.99999999999999645 ) ) ;
#3871=LINE ( 'NONE', #969, #1890 ) ;
#3872=EDGE_CURVE ( 'NONE', #4147, #819, #1061, .T. ) ;
#3873=VECTOR ( 'NONE', #4355, 1000.000000000000000 ) ;
#3890=CIRCLE ( 'NONE', #4575, 6.499999999999988454 ) ;
#3901=EDGE_LOOP ( 'NONE', ( #177, #1483, #1770, #1678 ) ) ;
#3915=LINE ( 'NONE', #1069, #3461 ) ;
#3921=EDGE_CURVE ( 'NONE', #3821, #1397, #4179, .T. ) ;
#3932=CARTESIAN_POINT ( 'NONE',  ( -25.00000000000000000, 610.0000000000000000, 24.99999999999999645 ) ) ;
#3958=FACE_OUTER_BOUND ( 'NONE', #2837, .T. ) ;
#3969=ORIENTED_EDGE ( 'NONE', *, *, #1718, .F. ) ;
#3986=VECTOR ( 'NONE', #2094, 1000.000000000000000 ) ;
#4004=CARTESIAN_POINT ( 'NONE',  ( -30.00000000000000355, 10.00000000000000000, -2.081668171172168908E-15 ) ) ;
#4026=VERTEX_POINT ( 'NONE', #4351 ) ;
#4028=VERTEX_POINT ( 'NONE', #257 ) ;
#4034=DIRECTION ( 'NONE',  ( -1.000000000000000000, 0.000000000000000000, 0.000000000000000000 ) ) ;
#4035=ORIENTED_EDGE ( 'NONE', *, *, #5360, .F. ) ;
#4050=ADVANCED_FACE ( 'NONE', ( #1105 ), #4772, .F. ) ;
#4056=ORIENTED_EDGE ( 'NONE', *, *, #4401, .F. ) ;
#4059=FACE_BOUND ( 'NONE', #2086, .T. ) ;
#4092=DIRECTION ( 'NONE',  ( -0.000000000000000000, -0.000000000000000000, 1.000000000000000000 ) ) ;
#4094=LINE ( 'NONE', #5363, #2688 ) ;
#4108=DIRECTION ( 'NONE',  ( 1.000000000000000000, 0.000000000000000000, 0.000000000000000000 ) ) ;
#4115=CARTESIAN_POINT ( 'NONE',  ( 25.00000000000000000, 610.0000000000000000, -25.00000000000000000 ) ) ;
#4133=PRODUCT_DEFINITION ( 'UNKNOWN', '', #840, #2824 ) ;
#4134=PLANE ( 'NONE',  #1101 ) ;
#4137=ORIENTED_EDGE ( 'NONE', *, *, #1066, .F. ) ;
#4138=CARTESIAN_POINT ( 'NONE',  ( -6.499999999999984901, 35.00000000000000000, 30.00000000000000711 ) ) ;
#4139=CARTESIAN_POINT ( 'NONE',  ( 6.499999999999981348, 35.00000000000000000, -25.00000000000000000 ) ) ;
#4142=ORIENTED_EDGE ( 'NONE', *, *, #3506, .T. ) ;
#4145=DIRECTION ( 'NONE',  ( 1.000000000000000000, 0.000000000000000000, 2.081668171172168513E-16 ) ) ;
#4147=VERTEX_POINT ( 'NONE', #1074 ) ;
#4151=VECTOR ( 'NONE', #505, 1000.000000000000000 ) ;
#4154=AXIS2_PLACEMENT_3D ( 'NONE', #2434, #5290, #769 ) ;
#4163=EDGE_CURVE ( 'NONE', #1969, #1397, #3174, .T. ) ;
#4179=LINE ( 'NONE', #5018, #3986 ) ;
#4188=ORIENTED_EDGE ( 'NONE', *, *, #4218, .F. ) ;
#4191=FACE_BOUND ( 'NONE', #1478, .T. ) ;
#4218=EDGE_CURVE ( 'NONE', #966, #1510, #4094, .T. ) ;
#4219=SURFACE_SIDE_STYLE ('',( #5011 ) ) ;
#4234=DIRECTION ( 'NONE',  ( -6.938893903907228378E-17, 0.000000000000000000, 1.000000000000000000 ) ) ;
#4242=( NAMED_UNIT ( * ) PLANE_ANGLE_UNIT ( ) SI_UNIT ( $, .RADIAN. ) );
#4249=DIRECTION ( 'NONE',  ( 1.000000000000000000, 0.000000000000000000, 0.000000000000000000 ) ) ;
#4251=AXIS2_PLACEMENT_3D ( 'NONE', #2319, #299, #1903 ) ;
#4252=ADVANCED_FACE ( 'NONE', ( #5339 ), #4948, .F. ) ;
#4253=ORIENTED_EDGE ( 'NONE', *, *, #1905, .F. ) ;
#4261=VERTEX_POINT ( 'NONE', #4139 ) ;
#4277=MECHANICAL_DESIGN_GEOMETRIC_PRESENTATION_REPRESENTATION('',(#1750),#1665);
#4281=CARTESIAN_POINT ( 'NONE',  ( 25.00000000000000000, 10.00000000000000000, 25.00000000000000711 ) ) ;
#4286=ADVANCED_BREP_SHAPE_REPRESENTATION ( '', ( #104, #4154 ), #3189 ) ;
#4287=DIRECTION ( 'NONE',  ( 0.000000000000000000, -0.000000000000000000, 1.000000000000000000 ) ) ;
#4291=LINE ( 'NONE', #4631, #4151 ) ;
#4302=CARTESIAN_POINT ( 'NONE',  ( -24.99999999999999645, 610.0000000000000000, -25.00000000000000000 ) ) ;
#4315=CARTESIAN_POINT ( 'NONE',  ( 30.00000000000000355, 610.0000000000000000, -30.00000000000000355 ) ) ;
#4330=FACE_OUTER_BOUND ( 'NONE', #3268, .T. ) ;
#4338=AXIS2_PLACEMENT_3D ( 'NONE', #5298, #4902, #776 ) ;
#4343=ADVANCED_FACE ( 'NONE', ( #4191, #3864 ), #1697, .T. ) ;
#4345=PLANE ( 'NONE',  #1688 ) ;
#4349=CARTESIAN_POINT ( 'NONE',  ( 25.00000000000000000, 610.0000000000000000, 25.00000000000000711 ) ) ;
#4351=CARTESIAN_POINT ( 'NONE',  ( -25.00000000000000000, 10.00000000000000000, 24.99999999999999645 ) ) ;
#4355=DIRECTION ( 'NONE',  ( -6.938893903907228378E-17, 0.000000000000000000, 1.000000000000000000 ) ) ;
#4360=CARTESIAN_POINT ( 'NONE',  ( 25.00000000000000000, 10.00000000000000000, 25.00000000000000711 ) ) ;
#4363=VERTEX_POINT ( 'NONE', #2166 ) ;
#4371=DIRECTION ( 'NONE',  ( -1.000000000000000000, 0.000000000000000000, 0.000000000000000000 ) ) ;
#4393=LINE ( 'NONE', #659, #761 ) ;
#4401=EDGE_CURVE ( 'NONE', #4261, #2639, #4415, .T. ) ;
#4411=CARTESIAN_POINT ( 'NONE',  ( 25.00000000000000000, 610.0000000000000000, 25.00000000000000711 ) ) ;
#4415=CIRCLE ( 'NONE', #502, 6.499999999999983125 ) ;
#4431=DIRECTION ( 'NONE',  ( -0.000000000000000000, -0.000000000000000000, 1.000000000000000000 ) ) ;
#4432=EDGE_CURVE ( 'NONE', #1397, #966, #3092, .T. ) ;
#4449=ORIENTED_EDGE ( 'NONE', *, *, #2743, .F. ) ;
#4454=VERTEX_POINT ( 'NONE', #1049 ) ;
#4496=LINE ( 'NONE', #5326, #3475 ) ;
#4512=VERTEX_POINT ( 'NONE', #1468 ) ;
#4525=EDGE_LOOP ( 'NONE', ( #1657, #2588 ) ) ;
#4544=CARTESIAN_POINT ( 'NONE',  ( -1.676835913137321903E-15, 35.00000000000000000, 25.00000000000000000 ) ) ;
#4550=PLANE ( 'NONE',  #1619 ) ;
#4552=LINE ( 'NONE', #3424, #3820 ) ;
#4557=LINE ( 'NONE', #4138, #652 ) ;
#4575=AXIS2_PLACEMENT_3D ( 'NONE', #858, #64, #2918 ) ;
#4584=ADVANCED_FACE ( 'NONE', ( #1410 ), #4737, .T. ) ;
#4596=( NAMED_UNIT ( * ) SI_UNIT ( $, .STERADIAN. ) SOLID_ANGLE_UNIT ( ) );
#4607=CARTESIAN_POINT ( 'NONE',  ( 25.00000000000000000, 610.0000000000000000, -25.00000000000000000 ) ) ;
#4616=ORIENTED_EDGE ( 'NONE', *, *, #3430, .T. ) ;
#4631=CARTESIAN_POINT ( 'NONE',  ( 6.499999999999981348, 35.00000000000000000, 30.00000000000000711 ) ) ;
#4642=LINE ( 'NONE', #1758, #1414 ) ;
#4643=DIRECTION ( 'NONE',  ( 1.000000000000000000, 0.000000000000000000, 0.000000000000000000 ) ) ;
#4668=CIRCLE ( 'NONE', #4338, 6.499999999999983125 ) ;
#4677=DIRECTION ( 'NONE',  ( 2.081668171172168513E-16, 0.000000000000000000, -1.000000000000000000 ) ) ;
#4682=CARTESIAN_POINT ( 'NONE',  ( 0.000000000000000000, 10.00000000000000000, 0.000000000000000000 ) ) ;
#4694=EDGE_CURVE ( 'NONE', #3498, #1075, #722, .T. ) ;
#4707=DIRECTION ( 'NONE',  ( 0.000000000000000000, 0.000000000000000000, -1.000000000000000000 ) ) ;
#4719=VERTEX_POINT ( 'NONE', #2184 ) ;
#4722=ORIENTED_EDGE ( 'NONE', *, *, #2387, .F. ) ;
#4737=PLANE ( 'NONE',  #3305 ) ;
#4751=EDGE_CURVE ( 'NONE', #5225, #4147, #4552, .T. ) ;
#4757=DIRECTION ( 'NONE',  ( 0.000000000000000000, 0.000000000000000000, -1.000000000000000000 ) ) ;
#4759=DIRECTION ( 'NONE',  ( -0.000000000000000000, -1.000000000000000000, -0.000000000000000000 ) ) ;
#4769=DIRECTION ( 'NONE',  ( -6.938893903907228378E-17, 0.000000000000000000, 1.000000000000000000 ) ) ;
#4772=CYLINDRICAL_SURFACE ( 'NONE', #1283, 6.499999999999993783 ) ;
#4775=ORIENTED_EDGE ( 'NONE', *, *, #3506, .F. ) ;
#4779=ORIENTED_EDGE ( 'NONE', *, *, #3921, .T. ) ;
#4780=DIRECTION ( 'NONE',  ( -1.000000000000000000, 0.000000000000000000, 0.000000000000000000 ) ) ;
#4782=VERTEX_POINT ( 'NONE', #4995 ) ;
#4789=VERTEX_POINT ( 'NONE', #4607 ) ;
#4799=DIRECTION ( 'NONE',  ( -0.000000000000000000, -0.000000000000000000, 1.000000000000000000 ) ) ;
#4800=EDGE_CURVE ( 'NONE', #4789, #5225, #65, .T. ) ;
#4829=MECHANICAL_DESIGN_GEOMETRIC_PRESENTATION_REPRESENTATION('',(#3627),#401);
#4831=CARTESIAN_POINT ( 'NONE',  ( 0.000000000000000000, 10.00000000000000000, -30.00000000000000355 ) ) ;
#4832=VERTEX_POINT ( 'NONE', #1872 ) ;
#4839=CARTESIAN_POINT ( 'NONE',  ( -30.00000000000000355, 610.0000000000000000, 30.00000000000000000 ) ) ;
#4851=FACE_BOUND ( 'NONE', #4525, .T. ) ;
#4865=FACE_BOUND ( 'NONE', #1995, .T. ) ;
#4878=EDGE_CURVE ( 'NONE', #1204, #2454, #3115, .T. ) ;
#4894=ORIENTED_EDGE ( 'NONE', *, *, #3142, .F. ) ;
#4902=DIRECTION ( 'NONE',  ( 0.000000000000000000, -0.000000000000000000, 1.000000000000000000 ) ) ;
#4919=EDGE_LOOP ( 'NONE', ( #169, #1054, #445, #4035 ) ) ;
#4927=VECTOR ( 'NONE', #1823, 1000.000000000000000 ) ;
#4947=DIRECTION ( 'NONE',  ( -0.000000000000000000, -1.000000000000000000, -0.000000000000000000 ) ) ;
#4948=PLANE ( 'NONE',  #3633 ) ;
#4954=ADVANCED_FACE ( 'NONE', ( #2290 ), #3553, .F. ) ;
#4973=EDGE_CURVE ( 'NONE', #4782, #1075, #2694, .T. ) ;
#4976=DIRECTION ( 'NONE',  ( -0.000000000000000000, -0.000000000000000000, 1.000000000000000000 ) ) ;
#4995=CARTESIAN_POINT ( 'NONE',  ( 6.499999999999988454, 570.0000000000000000, 30.00000000000000711 ) ) ;
#4999=ORIENTED_EDGE ( 'NONE', *, *, #1718, .T. ) ;
#5011=SURFACE_STYLE_FILL_AREA ( #845 ) ;
#5018=CARTESIAN_POINT ( 'NONE',  ( -30.00000000000000000, 610.0000000000000000, -30.00000000000000355 ) ) ;
#5030=CIRCLE ( 'NONE', #2679, 6.499999999999983125 ) ;
#5044=CARTESIAN_POINT ( 'NONE',  ( -6.499999999999988454, 570.0000000000000000, 30.00000000000000711 ) ) ;
#5061=APPLICATION_CONTEXT ( 'automotive_design' ) ;
#5071=EDGE_CURVE ( 'NONE', #4512, #2280, #4496, .T. ) ;
#5072=EDGE_CURVE ( 'NONE', #4832, #1591, #4668, .T. ) ;
#5104=VECTOR ( 'NONE', #2989, 1000.000000000000000 ) ;
#5106=FACE_OUTER_BOUND ( 'NONE', #2189, .T. ) ;
#5124=ORIENTED_EDGE ( 'NONE', *, *, #1066, .T. ) ;
#5127=LINE ( 'NONE', #134, #494 ) ;
#5135=CARTESIAN_POINT ( 'NONE',  ( -6.499999999999993783, 570.0000000000000000, 25.00000000000000000 ) ) ;
#5152=DIRECTION ( 'NONE',  ( -0.000000000000000000, -0.000000000000000000, 1.000000000000000000 ) ) ;
#5156=CARTESIAN_POINT ( 'NONE',  ( 30.00000000000000355, 10.00000000000000000, 30.00000000000001066 ) ) ;
#5158=DIRECTION ( 'NONE',  ( -0.000000000000000000, -1.000000000000000000, -0.000000000000000000 ) ) ;
#5162=EDGE_CURVE ( 'NONE', #676, #4719, #57, .T. ) ;
#5174=ORIENTED_EDGE ( 'NONE', *, *, #2566, .F. ) ;
#5197=VECTOR ( 'NONE', #4757, 1000.000000000000000 ) ;
#5214=EDGE_CURVE ( 'NONE', #819, #3218, #3871, .T. ) ;
#5225=VERTEX_POINT ( 'NONE', #4302 ) ;
#5229=CYLINDRICAL_SURFACE ( 'NONE', #3801, 6.499999999999993783 ) ;
#5245=EDGE_LOOP ( 'NONE', ( #5365, #635, #3149, #5174 ) ) ;
#5259=VECTOR ( 'NONE', #1038, 1000.000000000000000 ) ;
#5272=ORIENTED_EDGE ( 'NONE', *, *, #709, .T. ) ;
#5277=CARTESIAN_POINT ( 'NONE',  ( -6.499999999999993783, 570.0000000000000000, 30.00000000000000711 ) ) ;
#5279=CARTESIAN_POINT ( 'NONE',  ( -6.499999999999991118, 35.00000000000000000, 30.00000000000000711 ) ) ;
#5288=FACE_OUTER_BOUND ( 'NONE', #3901, .T. ) ;
#5290=DIRECTION ( 'NONE',  ( 0.000000000000000000, 0.000000000000000000, 1.000000000000000000 ) ) ;
#5298=CARTESIAN_POINT ( 'NONE',  ( -1.676835913137321903E-15, 35.00000000000000000, -30.00000000000000711 ) ) ;
#5305=ORIENTED_EDGE ( 'NONE', *, *, #4973, .T. ) ;
#5322=ORIENTED_EDGE ( 'NONE', *, *, #4800, .T. ) ;
#5326=CARTESIAN_POINT ( 'NONE',  ( -24.99999999999999645, 10.00000000000000000, -25.00000000000000000 ) ) ;
#5333=DIRECTION ( 'NONE',  ( 2.081668171172168513E-16, 0.000000000000000000, -1.000000000000000000 ) ) ;
#5339=FACE_OUTER_BOUND ( 'NONE', #851, .T. ) ;
#5360=EDGE_CURVE ( 'NONE', #4363, #4782, #3634, .T. ) ;
#5363=CARTESIAN_POINT ( 'NONE',  ( -6.245004513516506329E-15, 10.00000000000000000, 30.00000000000000711 ) ) ;
#5364=AXIS2_PLACEMENT_3D ( 'NONE', #554, #939, #4249 ) ;
#5365=ORIENTED_EDGE ( 'NONE', *, *, #1021, .F. ) ;
#5371=DIRECTION ( 'NONE',  ( 1.000000000000000000, 0.000000000000000000, 0.000000000000000000 ) ) ;
#5383=ADVANCED_FACE ( 'NONE', ( #293 ), #5229, .F. ) ;
#5434=COLOUR_RGB('Off White',0.89,0.88,0.83);
#5435=FILL_AREA_STYLE_COLOUR('',#5434);
#5436=FILL_AREA_STYLE('',(#5435));
#5437=SURFACE_STYLE_FILL_AREA(#5436);
#5438=SURFACE_SIDE_STYLE('',(#5437));
#5439=SURFACE_STYLE_USAGE(.BOTH.,#5438);
#5440=PRESENTATION_STYLE_ASSIGNMENT((#5439));
ENDSEC;
END-ISO-10303-21;
